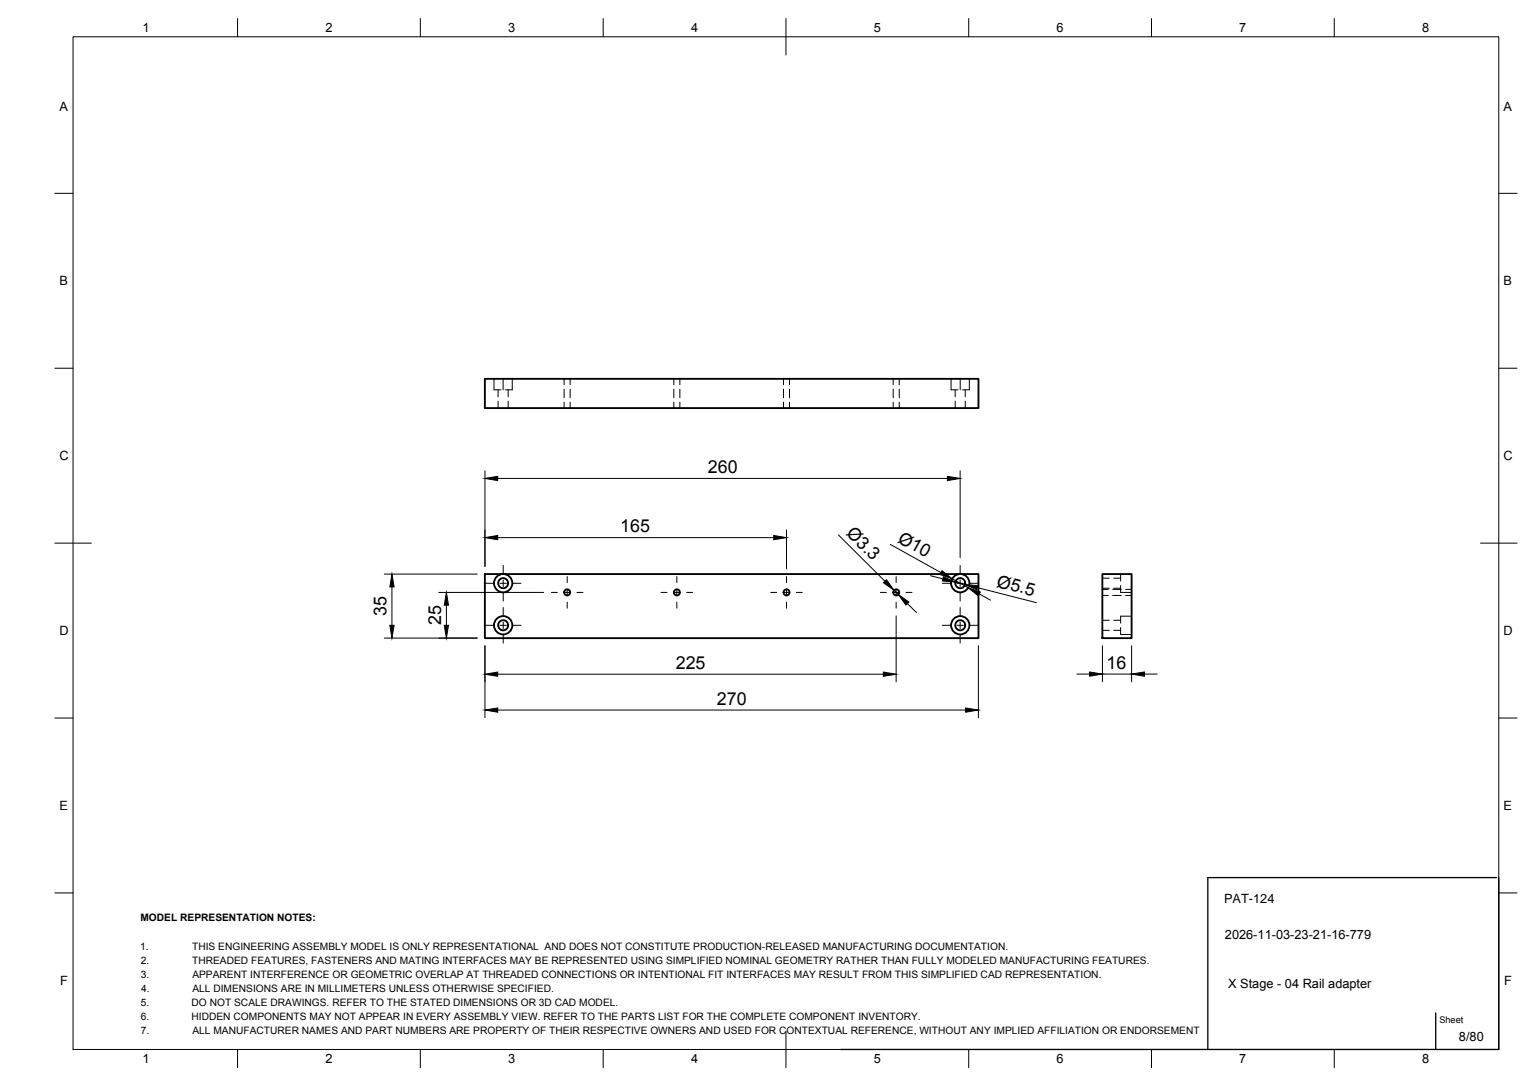
ISO-10303-21;
HEADER;
/* Generated by software containing ST-Developer
 * from STEP Tools, Inc. (www.steptools.com) 
 */

FILE_DESCRIPTION(
/* description */ ('XY cross-slide table'),
/* implementation_level */ '2;1');

FILE_NAME(
/* name */ 'X Stage - 04 Rail adapter.step',
/* time_stamp */ '2026-10-28T03:22:46-07:00',
/* author */ (''),
/* organization */ (''),
/* preprocessor_version */ 'ST-DEVELOPER v20.2',
/* originating_system */ 'Autodesk Translation Framework v15.17.0.0',
/* authorisation */ '');

FILE_SCHEMA (('AUTOMOTIVE_DESIGN { 1 0 10303 214 3 1 1 }'));
ENDSEC;

DATA;
#10=MECHANICAL_DESIGN_GEOMETRIC_PRESENTATION_REPRESENTATION('',(#1673),#62984);
#1507=SHAPE_REPRESENTATION_RELATIONSHIP('SRR','None',#63355,#1590);
#1590=ADVANCED_BREP_SHAPE_REPRESENTATION('',(#1786),#62892);
#1673=STYLED_ITEM('',(#63898),#1786);
#1786=MANIFOLD_SOLID_BREP('Body1',#22967);
#1907=FACE_BOUND('',#4239,.T.);
#1908=FACE_BOUND('',#4242,.T.);
#1909=FACE_BOUND('',#4245,.T.);
#1910=FACE_BOUND('',#4248,.T.);
#1911=FACE_BOUND('',#4250,.T.);
#1912=FACE_BOUND('',#4251,.T.);
#1913=FACE_BOUND('',#4252,.T.);
#1914=FACE_BOUND('',#4253,.T.);
#1915=FACE_BOUND('',#4254,.T.);
#1916=FACE_BOUND('',#4255,.T.);
#1917=FACE_BOUND('',#4265,.T.);
#1918=FACE_BOUND('',#4266,.T.);
#1919=FACE_BOUND('',#4267,.T.);
#1920=FACE_BOUND('',#4268,.T.);
#1921=FACE_BOUND('',#4269,.T.);
#1922=FACE_BOUND('',#4270,.T.);
#1923=FACE_BOUND('',#4271,.T.);
#1924=FACE_BOUND('',#4272,.T.);
#2314=PLANE('',#24076);
#2315=PLANE('',#24081);
#2316=PLANE('',#24086);
#2317=PLANE('',#24091);
#2318=PLANE('',#24093);
#2319=PLANE('',#24102);
#2320=PLANE('',#24103);
#2321=PLANE('',#24104);
#2322=PLANE('',#24105);
#2323=PLANE('',#24106);
#2897=FACE_OUTER_BOUND('',#4231,.T.);
#2898=FACE_OUTER_BOUND('',#4232,.T.);
#2899=FACE_OUTER_BOUND('',#4233,.T.);
#2900=FACE_OUTER_BOUND('',#4234,.T.);
#2901=FACE_OUTER_BOUND('',#4235,.T.);
#2902=FACE_OUTER_BOUND('',#4236,.T.);
#2903=FACE_OUTER_BOUND('',#4237,.T.);
#2904=FACE_OUTER_BOUND('',#4238,.T.);
#2905=FACE_OUTER_BOUND('',#4240,.T.);
#2906=FACE_OUTER_BOUND('',#4241,.T.);
#2907=FACE_OUTER_BOUND('',#4243,.T.);
#2908=FACE_OUTER_BOUND('',#4244,.T.);
#2909=FACE_OUTER_BOUND('',#4246,.T.);
#2910=FACE_OUTER_BOUND('',#4247,.T.);
#2911=FACE_OUTER_BOUND('',#4249,.T.);
#2912=FACE_OUTER_BOUND('',#4256,.T.);
#2913=FACE_OUTER_BOUND('',#4257,.T.);
#2914=FACE_OUTER_BOUND('',#4258,.T.);
#2915=FACE_OUTER_BOUND('',#4259,.T.);
#2916=FACE_OUTER_BOUND('',#4260,.T.);
#2917=FACE_OUTER_BOUND('',#4261,.T.);
#2918=FACE_OUTER_BOUND('',#4262,.T.);
#2919=FACE_OUTER_BOUND('',#4263,.T.);
#2920=FACE_OUTER_BOUND('',#4264,.T.);
#4231=EDGE_LOOP('',(#15036,#15037,#15038,#15039));
#4232=EDGE_LOOP('',(#15040,#15041,#15042,#15043));
#4233=EDGE_LOOP('',(#15044,#15045,#15046,#15047));
#4234=EDGE_LOOP('',(#15048,#15049,#15050,#15051));
#4235=EDGE_LOOP('',(#15052,#15053,#15054,#15055));
#4236=EDGE_LOOP('',(#15056,#15057,#15058,#15059));
#4237=EDGE_LOOP('',(#15060,#15061,#15062,#15063));
#4238=EDGE_LOOP('',(#15064));
#4239=EDGE_LOOP('',(#15065));
#4240=EDGE_LOOP('',(#15066,#15067,#15068,#15069));
#4241=EDGE_LOOP('',(#15070,#15071));
#4242=EDGE_LOOP('',(#15072));
#4243=EDGE_LOOP('',(#15073,#15074,#15075,#15076));
#4244=EDGE_LOOP('',(#15077));
#4245=EDGE_LOOP('',(#15078));
#4246=EDGE_LOOP('',(#15079,#15080,#15081,#15082));
#4247=EDGE_LOOP('',(#15083,#15084));
#4248=EDGE_LOOP('',(#15085));
#4249=EDGE_LOOP('',(#15086,#15087,#15088,#15089,#15090,#15091,#15092,#15093,
#15094,#15095));
#4250=EDGE_LOOP('',(#15096));
#4251=EDGE_LOOP('',(#15097));
#4252=EDGE_LOOP('',(#15098));
#4253=EDGE_LOOP('',(#15099));
#4254=EDGE_LOOP('',(#15100));
#4255=EDGE_LOOP('',(#15101));
#4256=EDGE_LOOP('',(#15102,#15103,#15104,#15105));
#4257=EDGE_LOOP('',(#15106,#15107,#15108,#15109));
#4258=EDGE_LOOP('',(#15110,#15111,#15112,#15113));
#4259=EDGE_LOOP('',(#15114,#15115,#15116,#15117));
#4260=EDGE_LOOP('',(#15118,#15119,#15120,#15121,#15122,#15123,#15124,#15125,
#15126,#15127));
#4261=EDGE_LOOP('',(#15128,#15129,#15130,#15131));
#4262=EDGE_LOOP('',(#15132,#15133,#15134,#15135));
#4263=EDGE_LOOP('',(#15136,#15137,#15138,#15139));
#4264=EDGE_LOOP('',(#15140,#15141,#15142,#15143));
#4265=EDGE_LOOP('',(#15144));
#4266=EDGE_LOOP('',(#15145));
#4267=EDGE_LOOP('',(#15146));
#4268=EDGE_LOOP('',(#15147));
#4269=EDGE_LOOP('',(#15148));
#4270=EDGE_LOOP('',(#15149));
#4271=EDGE_LOOP('',(#15150));
#4272=EDGE_LOOP('',(#15151));
#5952=LINE('',#33018,#7439);
#5953=LINE('',#33022,#7440);
#5954=LINE('',#33027,#7441);
#5955=LINE('',#33031,#7442);
#5956=LINE('',#33037,#7443);
#5957=LINE('',#33043,#7444);
#5958=LINE('',#33049,#7445);
#5959=LINE('',#33055,#7446);
#5960=LINE('',#33061,#7447);
#5961=LINE('',#33068,#7448);
#5962=LINE('',#33077,#7449);
#5963=LINE('',#33084,#7450);
#5964=LINE('',#33092,#7451);
#5965=LINE('',#33094,#7452);
#5966=LINE('',#33096,#7453);
#5967=LINE('',#33097,#7454);
#5968=LINE('',#33098,#7455);
#5969=LINE('',#33099,#7456);
#5970=LINE('',#33103,#7457);
#5971=LINE('',#33107,#7458);
#5972=LINE('',#33111,#7459);
#5973=LINE('',#33115,#7460);
#5974=LINE('',#33119,#7461);
#5975=LINE('',#33120,#7462);
#5976=LINE('',#33121,#7463);
#5977=LINE('',#33124,#7464);
#5978=LINE('',#33125,#7465);
#5979=LINE('',#33128,#7466);
#5980=LINE('',#33129,#7467);
#5981=LINE('',#33131,#7468);
#7439=VECTOR('',#26619,0.5);
#7440=VECTOR('',#26622,1.);
#7441=VECTOR('',#26627,0.5);
#7442=VECTOR('',#26630,1.);
#7443=VECTOR('',#26637,0.164999999999999);
#7444=VECTOR('',#26644,0.164999999999999);
#7445=VECTOR('',#26651,0.165);
#7446=VECTOR('',#26658,0.164999999999999);
#7447=VECTOR('',#26665,0.5);
#7448=VECTOR('',#26676,1.);
#7449=VECTOR('',#26687,0.5);
#7450=VECTOR('',#26698,1.);
#7451=VECTOR('',#26707,1.);
#7452=VECTOR('',#26708,1.);
#7453=VECTOR('',#26709,1.);
#7454=VECTOR('',#26710,1.);
#7455=VECTOR('',#26711,1.);
#7456=VECTOR('',#26712,1.);
#7457=VECTOR('',#26717,0.274999999999999);
#7458=VECTOR('',#26722,0.275);
#7459=VECTOR('',#26727,0.275);
#7460=VECTOR('',#26732,0.274999999999999);
#7461=VECTOR('',#26735,1.);
#7462=VECTOR('',#26736,1.);
#7463=VECTOR('',#26737,1.);
#7464=VECTOR('',#26740,1.);
#7465=VECTOR('',#26741,1.);
#7466=VECTOR('',#26744,1.);
#7467=VECTOR('',#26745,1.);
#7468=VECTOR('',#26748,1.);
#8900=CIRCLE('',#24056,0.5);
#8901=CIRCLE('',#24057,0.5);
#8902=CIRCLE('',#24059,0.5);
#8903=CIRCLE('',#24060,0.5);
#8904=CIRCLE('',#24062,0.164999999999999);
#8905=CIRCLE('',#24063,0.164999999999999);
#8906=CIRCLE('',#24065,0.164999999999999);
#8907=CIRCLE('',#24066,0.164999999999999);
#8908=CIRCLE('',#24068,0.165);
#8909=CIRCLE('',#24069,0.165);
#8910=CIRCLE('',#24071,0.164999999999999);
#8911=CIRCLE('',#24072,0.164999999999999);
#8912=CIRCLE('',#24074,0.5);
#8913=CIRCLE('',#24075,0.5);
#8914=CIRCLE('',#24077,0.274999999999999);
#8915=CIRCLE('',#24079,0.5);
#8916=CIRCLE('',#24080,0.5);
#8917=CIRCLE('',#24082,0.275);
#8918=CIRCLE('',#24084,0.5);
#8919=CIRCLE('',#24085,0.5);
#8920=CIRCLE('',#24087,0.275);
#8921=CIRCLE('',#24089,0.5);
#8922=CIRCLE('',#24090,0.5);
#8923=CIRCLE('',#24092,0.274999999999999);
#8924=CIRCLE('',#24095,0.274999999999999);
#8925=CIRCLE('',#24097,0.275);
#8926=CIRCLE('',#24099,0.275);
#8927=CIRCLE('',#24101,0.274999999999999);
#9817=VERTEX_POINT('',#33016);
#9818=VERTEX_POINT('',#33017);
#9819=VERTEX_POINT('',#33019);
#9820=VERTEX_POINT('',#33021);
#9821=VERTEX_POINT('',#33025);
#9822=VERTEX_POINT('',#33026);
#9823=VERTEX_POINT('',#33028);
#9824=VERTEX_POINT('',#33030);
#9825=VERTEX_POINT('',#33034);
#9826=VERTEX_POINT('',#33036);
#9827=VERTEX_POINT('',#33040);
#9828=VERTEX_POINT('',#33042);
#9829=VERTEX_POINT('',#33046);
#9830=VERTEX_POINT('',#33048);
#9831=VERTEX_POINT('',#33052);
#9832=VERTEX_POINT('',#33054);
#9833=VERTEX_POINT('',#33058);
#9834=VERTEX_POINT('',#33060);
#9835=VERTEX_POINT('',#33064);
#9836=VERTEX_POINT('',#33071);
#9837=VERTEX_POINT('',#33074);
#9838=VERTEX_POINT('',#33076);
#9839=VERTEX_POINT('',#33080);
#9840=VERTEX_POINT('',#33087);
#9841=VERTEX_POINT('',#33090);
#9842=VERTEX_POINT('',#33091);
#9843=VERTEX_POINT('',#33093);
#9844=VERTEX_POINT('',#33095);
#9845=VERTEX_POINT('',#33101);
#9846=VERTEX_POINT('',#33105);
#9847=VERTEX_POINT('',#33109);
#9848=VERTEX_POINT('',#33113);
#9849=VERTEX_POINT('',#33117);
#9850=VERTEX_POINT('',#33118);
#9851=VERTEX_POINT('',#33123);
#9852=VERTEX_POINT('',#33127);
#11902=EDGE_CURVE('',#9817,#9818,#5952,.T.);
#11903=EDGE_CURVE('',#9819,#9817,#8900,.T.);
#11904=EDGE_CURVE('',#9819,#9820,#5953,.T.);
#11905=EDGE_CURVE('',#9818,#9820,#8901,.T.);
#11906=EDGE_CURVE('',#9821,#9822,#5954,.T.);
#11907=EDGE_CURVE('',#9823,#9821,#8902,.T.);
#11908=EDGE_CURVE('',#9823,#9824,#5955,.T.);
#11909=EDGE_CURVE('',#9822,#9824,#8903,.T.);
#11910=EDGE_CURVE('',#9825,#9825,#8904,.T.);
#11911=EDGE_CURVE('',#9825,#9826,#5956,.T.);
#11912=EDGE_CURVE('',#9826,#9826,#8905,.T.);
#11913=EDGE_CURVE('',#9827,#9827,#8906,.T.);
#11914=EDGE_CURVE('',#9827,#9828,#5957,.T.);
#11915=EDGE_CURVE('',#9828,#9828,#8907,.T.);
#11916=EDGE_CURVE('',#9829,#9829,#8908,.T.);
#11917=EDGE_CURVE('',#9829,#9830,#5958,.T.);
#11918=EDGE_CURVE('',#9830,#9830,#8909,.T.);
#11919=EDGE_CURVE('',#9831,#9831,#8910,.T.);
#11920=EDGE_CURVE('',#9831,#9832,#5959,.T.);
#11921=EDGE_CURVE('',#9832,#9832,#8911,.T.);
#11922=EDGE_CURVE('',#9833,#9833,#8912,.T.);
#11923=EDGE_CURVE('',#9833,#9834,#5960,.T.);
#11924=EDGE_CURVE('',#9834,#9834,#8913,.T.);
#11925=EDGE_CURVE('',#9835,#9835,#8914,.T.);
#11926=EDGE_CURVE('',#9824,#9822,#8915,.T.);
#11927=EDGE_CURVE('',#9823,#9824,#5961,.T.);
#11928=EDGE_CURVE('',#9821,#9823,#8916,.T.);
#11929=EDGE_CURVE('',#9836,#9836,#8917,.T.);
#11930=EDGE_CURVE('',#9837,#9837,#8918,.T.);
#11931=EDGE_CURVE('',#9837,#9838,#5962,.T.);
#11932=EDGE_CURVE('',#9838,#9838,#8919,.T.);
#11933=EDGE_CURVE('',#9839,#9839,#8920,.T.);
#11934=EDGE_CURVE('',#9820,#9818,#8921,.T.);
#11935=EDGE_CURVE('',#9819,#9820,#5963,.T.);
#11936=EDGE_CURVE('',#9817,#9819,#8922,.T.);
#11937=EDGE_CURVE('',#9840,#9840,#8923,.T.);
#11938=EDGE_CURVE('',#9841,#9842,#5964,.T.);
#11939=EDGE_CURVE('',#9842,#9843,#5965,.T.);
#11940=EDGE_CURVE('',#9843,#9844,#5966,.T.);
#11941=EDGE_CURVE('',#9844,#9820,#5967,.T.);
#11942=EDGE_CURVE('',#9820,#9824,#5968,.T.);
#11943=EDGE_CURVE('',#9824,#9841,#5969,.T.);
#11944=EDGE_CURVE('',#9845,#9845,#8924,.T.);
#11945=EDGE_CURVE('',#9845,#9835,#5970,.T.);
#11946=EDGE_CURVE('',#9846,#9846,#8925,.T.);
#11947=EDGE_CURVE('',#9846,#9836,#5971,.T.);
#11948=EDGE_CURVE('',#9847,#9847,#8926,.T.);
#11949=EDGE_CURVE('',#9847,#9839,#5972,.T.);
#11950=EDGE_CURVE('',#9848,#9848,#8927,.T.);
#11951=EDGE_CURVE('',#9848,#9840,#5973,.T.);
#11952=EDGE_CURVE('',#9849,#9850,#5974,.T.);
#11953=EDGE_CURVE('',#9850,#9841,#5975,.T.);
#11954=EDGE_CURVE('',#9849,#9844,#5976,.T.);
#11955=EDGE_CURVE('',#9851,#9849,#5977,.T.);
#11956=EDGE_CURVE('',#9851,#9843,#5978,.T.);
#11957=EDGE_CURVE('',#9852,#9851,#5979,.T.);
#11958=EDGE_CURVE('',#9852,#9842,#5980,.T.);
#11959=EDGE_CURVE('',#9850,#9852,#5981,.T.);
#15036=ORIENTED_EDGE('',*,*,#11902,.F.);
#15037=ORIENTED_EDGE('',*,*,#11903,.F.);
#15038=ORIENTED_EDGE('',*,*,#11904,.T.);
#15039=ORIENTED_EDGE('',*,*,#11905,.F.);
#15040=ORIENTED_EDGE('',*,*,#11906,.F.);
#15041=ORIENTED_EDGE('',*,*,#11907,.F.);
#15042=ORIENTED_EDGE('',*,*,#11908,.T.);
#15043=ORIENTED_EDGE('',*,*,#11909,.F.);
#15044=ORIENTED_EDGE('',*,*,#11910,.F.);
#15045=ORIENTED_EDGE('',*,*,#11911,.T.);
#15046=ORIENTED_EDGE('',*,*,#11912,.F.);
#15047=ORIENTED_EDGE('',*,*,#11911,.F.);
#15048=ORIENTED_EDGE('',*,*,#11913,.F.);
#15049=ORIENTED_EDGE('',*,*,#11914,.T.);
#15050=ORIENTED_EDGE('',*,*,#11915,.F.);
#15051=ORIENTED_EDGE('',*,*,#11914,.F.);
#15052=ORIENTED_EDGE('',*,*,#11916,.F.);
#15053=ORIENTED_EDGE('',*,*,#11917,.T.);
#15054=ORIENTED_EDGE('',*,*,#11918,.F.);
#15055=ORIENTED_EDGE('',*,*,#11917,.F.);
#15056=ORIENTED_EDGE('',*,*,#11919,.F.);
#15057=ORIENTED_EDGE('',*,*,#11920,.T.);
#15058=ORIENTED_EDGE('',*,*,#11921,.F.);
#15059=ORIENTED_EDGE('',*,*,#11920,.F.);
#15060=ORIENTED_EDGE('',*,*,#11922,.F.);
#15061=ORIENTED_EDGE('',*,*,#11923,.T.);
#15062=ORIENTED_EDGE('',*,*,#11924,.F.);
#15063=ORIENTED_EDGE('',*,*,#11923,.F.);
#15064=ORIENTED_EDGE('',*,*,#11922,.T.);
#15065=ORIENTED_EDGE('',*,*,#11925,.F.);
#15066=ORIENTED_EDGE('',*,*,#11906,.T.);
#15067=ORIENTED_EDGE('',*,*,#11926,.F.);
#15068=ORIENTED_EDGE('',*,*,#11927,.F.);
#15069=ORIENTED_EDGE('',*,*,#11928,.F.);
#15070=ORIENTED_EDGE('',*,*,#11907,.T.);
#15071=ORIENTED_EDGE('',*,*,#11928,.T.);
#15072=ORIENTED_EDGE('',*,*,#11929,.F.);
#15073=ORIENTED_EDGE('',*,*,#11930,.F.);
#15074=ORIENTED_EDGE('',*,*,#11931,.T.);
#15075=ORIENTED_EDGE('',*,*,#11932,.F.);
#15076=ORIENTED_EDGE('',*,*,#11931,.F.);
#15077=ORIENTED_EDGE('',*,*,#11930,.T.);
#15078=ORIENTED_EDGE('',*,*,#11933,.F.);
#15079=ORIENTED_EDGE('',*,*,#11902,.T.);
#15080=ORIENTED_EDGE('',*,*,#11934,.F.);
#15081=ORIENTED_EDGE('',*,*,#11935,.F.);
#15082=ORIENTED_EDGE('',*,*,#11936,.F.);
#15083=ORIENTED_EDGE('',*,*,#11903,.T.);
#15084=ORIENTED_EDGE('',*,*,#11936,.T.);
#15085=ORIENTED_EDGE('',*,*,#11937,.F.);
#15086=ORIENTED_EDGE('',*,*,#11938,.T.);
#15087=ORIENTED_EDGE('',*,*,#11939,.T.);
#15088=ORIENTED_EDGE('',*,*,#11940,.T.);
#15089=ORIENTED_EDGE('',*,*,#11941,.T.);
#15090=ORIENTED_EDGE('',*,*,#11934,.T.);
#15091=ORIENTED_EDGE('',*,*,#11905,.T.);
#15092=ORIENTED_EDGE('',*,*,#11942,.T.);
#15093=ORIENTED_EDGE('',*,*,#11926,.T.);
#15094=ORIENTED_EDGE('',*,*,#11909,.T.);
#15095=ORIENTED_EDGE('',*,*,#11943,.T.);
#15096=ORIENTED_EDGE('',*,*,#11924,.T.);
#15097=ORIENTED_EDGE('',*,*,#11932,.T.);
#15098=ORIENTED_EDGE('',*,*,#11921,.T.);
#15099=ORIENTED_EDGE('',*,*,#11918,.T.);
#15100=ORIENTED_EDGE('',*,*,#11915,.T.);
#15101=ORIENTED_EDGE('',*,*,#11912,.T.);
#15102=ORIENTED_EDGE('',*,*,#11944,.F.);
#15103=ORIENTED_EDGE('',*,*,#11945,.T.);
#15104=ORIENTED_EDGE('',*,*,#11925,.T.);
#15105=ORIENTED_EDGE('',*,*,#11945,.F.);
#15106=ORIENTED_EDGE('',*,*,#11946,.F.);
#15107=ORIENTED_EDGE('',*,*,#11947,.T.);
#15108=ORIENTED_EDGE('',*,*,#11929,.T.);
#15109=ORIENTED_EDGE('',*,*,#11947,.F.);
#15110=ORIENTED_EDGE('',*,*,#11948,.F.);
#15111=ORIENTED_EDGE('',*,*,#11949,.T.);
#15112=ORIENTED_EDGE('',*,*,#11933,.T.);
#15113=ORIENTED_EDGE('',*,*,#11949,.F.);
#15114=ORIENTED_EDGE('',*,*,#11950,.F.);
#15115=ORIENTED_EDGE('',*,*,#11951,.T.);
#15116=ORIENTED_EDGE('',*,*,#11937,.T.);
#15117=ORIENTED_EDGE('',*,*,#11951,.F.);
#15118=ORIENTED_EDGE('',*,*,#11952,.T.);
#15119=ORIENTED_EDGE('',*,*,#11953,.T.);
#15120=ORIENTED_EDGE('',*,*,#11943,.F.);
#15121=ORIENTED_EDGE('',*,*,#11908,.F.);
#15122=ORIENTED_EDGE('',*,*,#11927,.T.);
#15123=ORIENTED_EDGE('',*,*,#11942,.F.);
#15124=ORIENTED_EDGE('',*,*,#11904,.F.);
#15125=ORIENTED_EDGE('',*,*,#11935,.T.);
#15126=ORIENTED_EDGE('',*,*,#11941,.F.);
#15127=ORIENTED_EDGE('',*,*,#11954,.F.);
#15128=ORIENTED_EDGE('',*,*,#11955,.T.);
#15129=ORIENTED_EDGE('',*,*,#11954,.T.);
#15130=ORIENTED_EDGE('',*,*,#11940,.F.);
#15131=ORIENTED_EDGE('',*,*,#11956,.F.);
#15132=ORIENTED_EDGE('',*,*,#11957,.T.);
#15133=ORIENTED_EDGE('',*,*,#11956,.T.);
#15134=ORIENTED_EDGE('',*,*,#11939,.F.);
#15135=ORIENTED_EDGE('',*,*,#11958,.F.);
#15136=ORIENTED_EDGE('',*,*,#11959,.T.);
#15137=ORIENTED_EDGE('',*,*,#11958,.T.);
#15138=ORIENTED_EDGE('',*,*,#11938,.F.);
#15139=ORIENTED_EDGE('',*,*,#11953,.F.);
#15140=ORIENTED_EDGE('',*,*,#11959,.F.);
#15141=ORIENTED_EDGE('',*,*,#11952,.F.);
#15142=ORIENTED_EDGE('',*,*,#11955,.F.);
#15143=ORIENTED_EDGE('',*,*,#11957,.F.);
#15144=ORIENTED_EDGE('',*,*,#11950,.T.);
#15145=ORIENTED_EDGE('',*,*,#11948,.T.);
#15146=ORIENTED_EDGE('',*,*,#11946,.T.);
#15147=ORIENTED_EDGE('',*,*,#11944,.T.);
#15148=ORIENTED_EDGE('',*,*,#11919,.T.);
#15149=ORIENTED_EDGE('',*,*,#11916,.T.);
#15150=ORIENTED_EDGE('',*,*,#11913,.T.);
#15151=ORIENTED_EDGE('',*,*,#11910,.T.);
#21050=CYLINDRICAL_SURFACE('',#24055,0.5);
#21051=CYLINDRICAL_SURFACE('',#24058,0.5);
#21052=CYLINDRICAL_SURFACE('',#24061,0.164999999999999);
#21053=CYLINDRICAL_SURFACE('',#24064,0.164999999999999);
#21054=CYLINDRICAL_SURFACE('',#24067,0.165);
#21055=CYLINDRICAL_SURFACE('',#24070,0.164999999999999);
#21056=CYLINDRICAL_SURFACE('',#24073,0.5);
#21057=CYLINDRICAL_SURFACE('',#24078,0.5);
#21058=CYLINDRICAL_SURFACE('',#24083,0.5);
#21059=CYLINDRICAL_SURFACE('',#24088,0.5);
#21060=CYLINDRICAL_SURFACE('',#24094,0.274999999999999);
#21061=CYLINDRICAL_SURFACE('',#24096,0.275);
#21062=CYLINDRICAL_SURFACE('',#24098,0.275);
#21063=CYLINDRICAL_SURFACE('',#24100,0.274999999999999);
#21678=ADVANCED_FACE('',(#2897),#21050,.F.);
#21679=ADVANCED_FACE('',(#2898),#21051,.F.);
#21680=ADVANCED_FACE('',(#2899),#21052,.F.);
#21681=ADVANCED_FACE('',(#2900),#21053,.F.);
#21682=ADVANCED_FACE('',(#2901),#21054,.F.);
#21683=ADVANCED_FACE('',(#2902),#21055,.F.);
#21684=ADVANCED_FACE('',(#2903),#21056,.F.);
#21685=ADVANCED_FACE('',(#2904,#1907),#2314,.T.);
#21686=ADVANCED_FACE('',(#2905),#21057,.F.);
#21687=ADVANCED_FACE('',(#2906,#1908),#2315,.T.);
#21688=ADVANCED_FACE('',(#2907),#21058,.F.);
#21689=ADVANCED_FACE('',(#2908,#1909),#2316,.T.);
#21690=ADVANCED_FACE('',(#2909),#21059,.F.);
#21691=ADVANCED_FACE('',(#2910,#1910),#2317,.T.);
#21692=ADVANCED_FACE('',(#2911,#1911,#1912,#1913,#1914,#1915,#1916),#2318,
 .T.);
#21693=ADVANCED_FACE('',(#2912),#21060,.F.);
#21694=ADVANCED_FACE('',(#2913),#21061,.F.);
#21695=ADVANCED_FACE('',(#2914),#21062,.F.);
#21696=ADVANCED_FACE('',(#2915),#21063,.F.);
#21697=ADVANCED_FACE('',(#2916),#2319,.T.);
#21698=ADVANCED_FACE('',(#2917),#2320,.T.);
#21699=ADVANCED_FACE('',(#2918),#2321,.T.);
#21700=ADVANCED_FACE('',(#2919),#2322,.T.);
#21701=ADVANCED_FACE('',(#2920,#1917,#1918,#1919,#1920,#1921,#1922,#1923,
#1924),#2323,.F.);
#22967=CLOSED_SHELL('',(#21678,#21679,#21680,#21681,#21682,#21683,#21684,
#21685,#21686,#21687,#21688,#21689,#21690,#21691,#21692,#21693,#21694,#21695,
#21696,#21697,#21698,#21699,#21700,#21701));
#24054=AXIS2_PLACEMENT_3D('',#33014,#26615,#26616);
#24055=AXIS2_PLACEMENT_3D('',#33015,#26617,#26618);
#24056=AXIS2_PLACEMENT_3D('',#33020,#26620,#26621);
#24057=AXIS2_PLACEMENT_3D('',#33023,#26623,#26624);
#24058=AXIS2_PLACEMENT_3D('',#33024,#26625,#26626);
#24059=AXIS2_PLACEMENT_3D('',#33029,#26628,#26629);
#24060=AXIS2_PLACEMENT_3D('',#33032,#26631,#26632);
#24061=AXIS2_PLACEMENT_3D('',#33033,#26633,#26634);
#24062=AXIS2_PLACEMENT_3D('',#33035,#26635,#26636);
#24063=AXIS2_PLACEMENT_3D('',#33038,#26638,#26639);
#24064=AXIS2_PLACEMENT_3D('',#33039,#26640,#26641);
#24065=AXIS2_PLACEMENT_3D('',#33041,#26642,#26643);
#24066=AXIS2_PLACEMENT_3D('',#33044,#26645,#26646);
#24067=AXIS2_PLACEMENT_3D('',#33045,#26647,#26648);
#24068=AXIS2_PLACEMENT_3D('',#33047,#26649,#26650);
#24069=AXIS2_PLACEMENT_3D('',#33050,#26652,#26653);
#24070=AXIS2_PLACEMENT_3D('',#33051,#26654,#26655);
#24071=AXIS2_PLACEMENT_3D('',#33053,#26656,#26657);
#24072=AXIS2_PLACEMENT_3D('',#33056,#26659,#26660);
#24073=AXIS2_PLACEMENT_3D('',#33057,#26661,#26662);
#24074=AXIS2_PLACEMENT_3D('',#33059,#26663,#26664);
#24075=AXIS2_PLACEMENT_3D('',#33062,#26666,#26667);
#24076=AXIS2_PLACEMENT_3D('',#33063,#26668,#26669);
#24077=AXIS2_PLACEMENT_3D('',#33065,#26670,#26671);
#24078=AXIS2_PLACEMENT_3D('',#33066,#26672,#26673);
#24079=AXIS2_PLACEMENT_3D('',#33067,#26674,#26675);
#24080=AXIS2_PLACEMENT_3D('',#33069,#26677,#26678);
#24081=AXIS2_PLACEMENT_3D('',#33070,#26679,#26680);
#24082=AXIS2_PLACEMENT_3D('',#33072,#26681,#26682);
#24083=AXIS2_PLACEMENT_3D('',#33073,#26683,#26684);
#24084=AXIS2_PLACEMENT_3D('',#33075,#26685,#26686);
#24085=AXIS2_PLACEMENT_3D('',#33078,#26688,#26689);
#24086=AXIS2_PLACEMENT_3D('',#33079,#26690,#26691);
#24087=AXIS2_PLACEMENT_3D('',#33081,#26692,#26693);
#24088=AXIS2_PLACEMENT_3D('',#33082,#26694,#26695);
#24089=AXIS2_PLACEMENT_3D('',#33083,#26696,#26697);
#24090=AXIS2_PLACEMENT_3D('',#33085,#26699,#26700);
#24091=AXIS2_PLACEMENT_3D('',#33086,#26701,#26702);
#24092=AXIS2_PLACEMENT_3D('',#33088,#26703,#26704);
#24093=AXIS2_PLACEMENT_3D('',#33089,#26705,#26706);
#24094=AXIS2_PLACEMENT_3D('',#33100,#26713,#26714);
#24095=AXIS2_PLACEMENT_3D('',#33102,#26715,#26716);
#24096=AXIS2_PLACEMENT_3D('',#33104,#26718,#26719);
#24097=AXIS2_PLACEMENT_3D('',#33106,#26720,#26721);
#24098=AXIS2_PLACEMENT_3D('',#33108,#26723,#26724);
#24099=AXIS2_PLACEMENT_3D('',#33110,#26725,#26726);
#24100=AXIS2_PLACEMENT_3D('',#33112,#26728,#26729);
#24101=AXIS2_PLACEMENT_3D('',#33114,#26730,#26731);
#24102=AXIS2_PLACEMENT_3D('',#33116,#26733,#26734);
#24103=AXIS2_PLACEMENT_3D('',#33122,#26738,#26739);
#24104=AXIS2_PLACEMENT_3D('',#33126,#26742,#26743);
#24105=AXIS2_PLACEMENT_3D('',#33130,#26746,#26747);
#24106=AXIS2_PLACEMENT_3D('',#33132,#26749,#26750);
#26615=DIRECTION('axis',(0.,0.,1.));
#26616=DIRECTION('refdir',(1.,0.,0.));
#26617=DIRECTION('center_axis',(0.,0.,1.));
#26618=DIRECTION('ref_axis',(1.,0.,0.));
#26619=DIRECTION('',(0.,0.,1.));
#26620=DIRECTION('center_axis',(0.,0.,1.));
#26621=DIRECTION('ref_axis',(1.,0.,0.));
#26622=DIRECTION('',(0.,0.,1.));
#26623=DIRECTION('center_axis',(0.,0.,-1.));
#26624=DIRECTION('ref_axis',(1.,0.,0.));
#26625=DIRECTION('center_axis',(0.,0.,1.));
#26626=DIRECTION('ref_axis',(1.,0.,0.));
#26627=DIRECTION('',(0.,0.,1.));
#26628=DIRECTION('center_axis',(0.,0.,1.));
#26629=DIRECTION('ref_axis',(1.,0.,0.));
#26630=DIRECTION('',(0.,0.,1.));
#26631=DIRECTION('center_axis',(0.,0.,-1.));
#26632=DIRECTION('ref_axis',(1.,0.,0.));
#26633=DIRECTION('center_axis',(0.,0.,1.));
#26634=DIRECTION('ref_axis',(1.,0.,0.));
#26635=DIRECTION('center_axis',(0.,0.,1.));
#26636=DIRECTION('ref_axis',(1.,0.,0.));
#26637=DIRECTION('',(0.,0.,1.));
#26638=DIRECTION('center_axis',(0.,0.,-1.));
#26639=DIRECTION('ref_axis',(1.,0.,0.));
#26640=DIRECTION('center_axis',(0.,0.,1.));
#26641=DIRECTION('ref_axis',(1.,0.,0.));
#26642=DIRECTION('center_axis',(0.,0.,1.));
#26643=DIRECTION('ref_axis',(1.,0.,0.));
#26644=DIRECTION('',(0.,0.,1.));
#26645=DIRECTION('center_axis',(0.,0.,-1.));
#26646=DIRECTION('ref_axis',(1.,0.,0.));
#26647=DIRECTION('center_axis',(0.,0.,1.));
#26648=DIRECTION('ref_axis',(1.,0.,0.));
#26649=DIRECTION('center_axis',(0.,0.,1.));
#26650=DIRECTION('ref_axis',(1.,0.,0.));
#26651=DIRECTION('',(0.,0.,1.));
#26652=DIRECTION('center_axis',(0.,0.,-1.));
#26653=DIRECTION('ref_axis',(1.,0.,0.));
#26654=DIRECTION('center_axis',(0.,0.,1.));
#26655=DIRECTION('ref_axis',(1.,0.,0.));
#26656=DIRECTION('center_axis',(0.,0.,1.));
#26657=DIRECTION('ref_axis',(1.,0.,0.));
#26658=DIRECTION('',(0.,0.,1.));
#26659=DIRECTION('center_axis',(0.,0.,-1.));
#26660=DIRECTION('ref_axis',(1.,0.,0.));
#26661=DIRECTION('center_axis',(0.,0.,1.));
#26662=DIRECTION('ref_axis',(1.,0.,0.));
#26663=DIRECTION('center_axis',(0.,0.,1.));
#26664=DIRECTION('ref_axis',(1.,0.,0.));
#26665=DIRECTION('',(0.,0.,1.));
#26666=DIRECTION('center_axis',(0.,0.,-1.));
#26667=DIRECTION('ref_axis',(1.,0.,0.));
#26668=DIRECTION('center_axis',(0.,0.,1.));
#26669=DIRECTION('ref_axis',(1.,0.,0.));
#26670=DIRECTION('center_axis',(0.,0.,1.));
#26671=DIRECTION('ref_axis',(1.,0.,0.));
#26672=DIRECTION('center_axis',(0.,0.,1.));
#26673=DIRECTION('ref_axis',(1.,0.,0.));
#26674=DIRECTION('center_axis',(0.,0.,-1.));
#26675=DIRECTION('ref_axis',(1.,0.,0.));
#26676=DIRECTION('',(0.,0.,1.));
#26677=DIRECTION('center_axis',(0.,0.,1.));
#26678=DIRECTION('ref_axis',(1.,0.,0.));
#26679=DIRECTION('center_axis',(0.,0.,1.));
#26680=DIRECTION('ref_axis',(1.,0.,0.));
#26681=DIRECTION('center_axis',(0.,0.,1.));
#26682=DIRECTION('ref_axis',(1.,0.,0.));
#26683=DIRECTION('center_axis',(0.,0.,1.));
#26684=DIRECTION('ref_axis',(1.,0.,0.));
#26685=DIRECTION('center_axis',(0.,0.,1.));
#26686=DIRECTION('ref_axis',(1.,0.,0.));
#26687=DIRECTION('',(0.,0.,1.));
#26688=DIRECTION('center_axis',(0.,0.,-1.));
#26689=DIRECTION('ref_axis',(1.,0.,0.));
#26690=DIRECTION('center_axis',(0.,0.,1.));
#26691=DIRECTION('ref_axis',(1.,0.,0.));
#26692=DIRECTION('center_axis',(0.,0.,1.));
#26693=DIRECTION('ref_axis',(1.,0.,0.));
#26694=DIRECTION('center_axis',(0.,0.,1.));
#26695=DIRECTION('ref_axis',(1.,0.,0.));
#26696=DIRECTION('center_axis',(0.,0.,-1.));
#26697=DIRECTION('ref_axis',(1.,0.,0.));
#26698=DIRECTION('',(0.,0.,1.));
#26699=DIRECTION('center_axis',(0.,0.,1.));
#26700=DIRECTION('ref_axis',(1.,0.,0.));
#26701=DIRECTION('center_axis',(0.,0.,1.));
#26702=DIRECTION('ref_axis',(1.,0.,0.));
#26703=DIRECTION('center_axis',(0.,0.,1.));
#26704=DIRECTION('ref_axis',(1.,0.,0.));
#26705=DIRECTION('center_axis',(0.,0.,1.));
#26706=DIRECTION('ref_axis',(1.,0.,0.));
#26707=DIRECTION('',(0.,-1.,0.));
#26708=DIRECTION('',(1.,0.,0.));
#26709=DIRECTION('',(0.,1.,0.));
#26710=DIRECTION('',(-1.,0.,0.));
#26711=DIRECTION('',(-1.,0.,0.));
#26712=DIRECTION('',(-1.,0.,0.));
#26713=DIRECTION('center_axis',(0.,0.,1.));
#26714=DIRECTION('ref_axis',(1.,0.,0.));
#26715=DIRECTION('center_axis',(0.,0.,1.));
#26716=DIRECTION('ref_axis',(1.,0.,0.));
#26717=DIRECTION('',(0.,0.,1.));
#26718=DIRECTION('center_axis',(0.,0.,1.));
#26719=DIRECTION('ref_axis',(1.,0.,0.));
#26720=DIRECTION('center_axis',(0.,0.,1.));
#26721=DIRECTION('ref_axis',(1.,0.,0.));
#26722=DIRECTION('',(0.,0.,1.));
#26723=DIRECTION('center_axis',(0.,0.,1.));
#26724=DIRECTION('ref_axis',(1.,0.,0.));
#26725=DIRECTION('center_axis',(0.,0.,1.));
#26726=DIRECTION('ref_axis',(1.,0.,0.));
#26727=DIRECTION('',(0.,0.,1.));
#26728=DIRECTION('center_axis',(0.,0.,1.));
#26729=DIRECTION('ref_axis',(1.,0.,0.));
#26730=DIRECTION('center_axis',(0.,0.,1.));
#26731=DIRECTION('ref_axis',(1.,0.,0.));
#26732=DIRECTION('',(0.,0.,1.));
#26733=DIRECTION('center_axis',(0.,1.,0.));
#26734=DIRECTION('ref_axis',(-1.,0.,0.));
#26735=DIRECTION('',(-1.,0.,0.));
#26736=DIRECTION('',(0.,0.,1.));
#26737=DIRECTION('',(0.,0.,1.));
#26738=DIRECTION('center_axis',(1.,0.,0.));
#26739=DIRECTION('ref_axis',(0.,1.,0.));
#26740=DIRECTION('',(0.,1.,0.));
#26741=DIRECTION('',(0.,0.,1.));
#26742=DIRECTION('center_axis',(0.,-1.,0.));
#26743=DIRECTION('ref_axis',(1.,0.,0.));
#26744=DIRECTION('',(1.,0.,0.));
#26745=DIRECTION('',(0.,0.,1.));
#26746=DIRECTION('center_axis',(-1.,0.,0.));
#26747=DIRECTION('ref_axis',(0.,-1.,0.));
#26748=DIRECTION('',(0.,-1.,0.));
#26749=DIRECTION('center_axis',(0.,0.,1.));
#26750=DIRECTION('ref_axis',(1.,0.,0.));
#33014=CARTESIAN_POINT('',(0.,0.,0.));
#33015=CARTESIAN_POINT('Origin',(26.,-5.5,2.2));
#33016=CARTESIAN_POINT('',(25.5,-5.5,2.2));
#33017=CARTESIAN_POINT('',(25.5,-5.5,2.8));
#33018=CARTESIAN_POINT('',(25.5,-5.5,2.2));
#33019=CARTESIAN_POINT('',(26.,-5.,2.2));
#33020=CARTESIAN_POINT('Origin',(26.,-5.5,2.2));
#33021=CARTESIAN_POINT('',(26.,-5.,2.8));
#33022=CARTESIAN_POINT('',(26.,-5.,2.2));
#33023=CARTESIAN_POINT('Origin',(26.,-5.5,2.8));
#33024=CARTESIAN_POINT('Origin',(1.,-5.5,2.2));
#33025=CARTESIAN_POINT('',(0.5,-5.5,2.2));
#33026=CARTESIAN_POINT('',(0.5,-5.5,2.8));
#33027=CARTESIAN_POINT('',(0.5,-5.5,2.2));
#33028=CARTESIAN_POINT('',(1.,-5.,2.2));
#33029=CARTESIAN_POINT('Origin',(1.,-5.5,2.2));
#33030=CARTESIAN_POINT('',(1.,-5.,2.8));
#33031=CARTESIAN_POINT('',(1.,-5.,2.2));
#33032=CARTESIAN_POINT('Origin',(1.,-5.5,2.8));
#33033=CARTESIAN_POINT('Origin',(16.5,-6.,1.1));
#33034=CARTESIAN_POINT('',(16.335,-6.,1.2));
#33035=CARTESIAN_POINT('Origin',(16.5,-6.,1.2));
#33036=CARTESIAN_POINT('',(16.335,-6.,2.8));
#33037=CARTESIAN_POINT('',(16.335,-6.,1.1));
#33038=CARTESIAN_POINT('Origin',(16.5,-6.,2.8));
#33039=CARTESIAN_POINT('Origin',(10.5,-6.,1.1));
#33040=CARTESIAN_POINT('',(10.335,-6.,1.2));
#33041=CARTESIAN_POINT('Origin',(10.5,-6.,1.2));
#33042=CARTESIAN_POINT('',(10.335,-6.,2.8));
#33043=CARTESIAN_POINT('',(10.335,-6.,1.1));
#33044=CARTESIAN_POINT('Origin',(10.5,-6.,2.8));
#33045=CARTESIAN_POINT('Origin',(4.5,-6.,1.1));
#33046=CARTESIAN_POINT('',(4.335,-6.,1.2));
#33047=CARTESIAN_POINT('Origin',(4.5,-6.,1.2));
#33048=CARTESIAN_POINT('',(4.335,-6.,2.8));
#33049=CARTESIAN_POINT('',(4.335,-6.,1.1));
#33050=CARTESIAN_POINT('Origin',(4.5,-6.,2.8));
#33051=CARTESIAN_POINT('Origin',(22.5,-6.,1.1));
#33052=CARTESIAN_POINT('',(22.335,-6.,1.2));
#33053=CARTESIAN_POINT('Origin',(22.5,-6.,1.2));
#33054=CARTESIAN_POINT('',(22.335,-6.,2.8));
#33055=CARTESIAN_POINT('',(22.335,-6.,1.1));
#33056=CARTESIAN_POINT('Origin',(22.5,-6.,2.8));
#33057=CARTESIAN_POINT('Origin',(26.,-7.8,2.2));
#33058=CARTESIAN_POINT('',(25.5,-7.8,2.2));
#33059=CARTESIAN_POINT('Origin',(26.,-7.8,2.2));
#33060=CARTESIAN_POINT('',(25.5,-7.8,2.8));
#33061=CARTESIAN_POINT('',(25.5,-7.8,2.2));
#33062=CARTESIAN_POINT('Origin',(26.,-7.8,2.8));
#33063=CARTESIAN_POINT('Origin',(26.,-7.8,2.2));
#33064=CARTESIAN_POINT('',(25.725,-7.8,2.2));
#33065=CARTESIAN_POINT('Origin',(26.,-7.8,2.2));
#33066=CARTESIAN_POINT('Origin',(1.,-5.5,2.2));
#33067=CARTESIAN_POINT('Origin',(1.,-5.5,2.8));
#33068=CARTESIAN_POINT('',(1.,-5.,2.2));
#33069=CARTESIAN_POINT('Origin',(1.,-5.5,2.2));
#33070=CARTESIAN_POINT('Origin',(1.,-5.5,2.2));
#33071=CARTESIAN_POINT('',(0.725,-5.5,2.2));
#33072=CARTESIAN_POINT('Origin',(1.,-5.5,2.2));
#33073=CARTESIAN_POINT('Origin',(1.,-7.8,2.2));
#33074=CARTESIAN_POINT('',(0.5,-7.8,2.2));
#33075=CARTESIAN_POINT('Origin',(1.,-7.8,2.2));
#33076=CARTESIAN_POINT('',(0.5,-7.8,2.8));
#33077=CARTESIAN_POINT('',(0.5,-7.8,2.2));
#33078=CARTESIAN_POINT('Origin',(1.,-7.8,2.8));
#33079=CARTESIAN_POINT('Origin',(1.,-7.8,2.2));
#33080=CARTESIAN_POINT('',(0.725,-7.8,2.2));
#33081=CARTESIAN_POINT('Origin',(1.,-7.8,2.2));
#33082=CARTESIAN_POINT('Origin',(26.,-5.5,2.2));
#33083=CARTESIAN_POINT('Origin',(26.,-5.5,2.8));
#33084=CARTESIAN_POINT('',(26.,-5.,2.2));
#33085=CARTESIAN_POINT('Origin',(26.,-5.5,2.2));
#33086=CARTESIAN_POINT('Origin',(26.,-5.5,2.2));
#33087=CARTESIAN_POINT('',(25.725,-5.5,2.2));
#33088=CARTESIAN_POINT('Origin',(26.,-5.5,2.2));
#33089=CARTESIAN_POINT('Origin',(13.5,-6.75,2.8));
#33090=CARTESIAN_POINT('',(0.,-5.,2.8));
#33091=CARTESIAN_POINT('',(0.,-8.5,2.8));
#33092=CARTESIAN_POINT('',(0.,-5.,2.8));
#33093=CARTESIAN_POINT('',(27.,-8.5,2.8));
#33094=CARTESIAN_POINT('',(0.,-8.5,2.8));
#33095=CARTESIAN_POINT('',(27.,-5.,2.8));
#33096=CARTESIAN_POINT('',(27.,-8.5,2.8));
#33097=CARTESIAN_POINT('',(27.,-5.,2.8));
#33098=CARTESIAN_POINT('',(27.,-5.,2.8));
#33099=CARTESIAN_POINT('',(27.,-5.,2.8));
#33100=CARTESIAN_POINT('Origin',(26.,-7.8,1.1));
#33101=CARTESIAN_POINT('',(25.725,-7.8,1.2));
#33102=CARTESIAN_POINT('Origin',(26.,-7.8,1.2));
#33103=CARTESIAN_POINT('',(25.725,-7.8,1.1));
#33104=CARTESIAN_POINT('Origin',(1.,-5.5,1.1));
#33105=CARTESIAN_POINT('',(0.725,-5.5,1.2));
#33106=CARTESIAN_POINT('Origin',(1.,-5.5,1.2));
#33107=CARTESIAN_POINT('',(0.725,-5.5,1.1));
#33108=CARTESIAN_POINT('Origin',(1.,-7.8,1.1));
#33109=CARTESIAN_POINT('',(0.725,-7.8,1.2));
#33110=CARTESIAN_POINT('Origin',(1.,-7.8,1.2));
#33111=CARTESIAN_POINT('',(0.725,-7.8,1.1));
#33112=CARTESIAN_POINT('Origin',(26.,-5.5,1.1));
#33113=CARTESIAN_POINT('',(25.725,-5.5,1.2));
#33114=CARTESIAN_POINT('Origin',(26.,-5.5,1.2));
#33115=CARTESIAN_POINT('',(25.725,-5.5,1.1));
#33116=CARTESIAN_POINT('Origin',(27.,-5.,1.2));
#33117=CARTESIAN_POINT('',(27.,-5.,1.2));
#33118=CARTESIAN_POINT('',(0.,-5.,1.2));
#33119=CARTESIAN_POINT('',(27.,-5.,1.2));
#33120=CARTESIAN_POINT('',(0.,-5.,1.2));
#33121=CARTESIAN_POINT('',(27.,-5.,1.2));
#33122=CARTESIAN_POINT('Origin',(27.,-8.5,1.2));
#33123=CARTESIAN_POINT('',(27.,-8.5,1.2));
#33124=CARTESIAN_POINT('',(27.,-8.5,1.2));
#33125=CARTESIAN_POINT('',(27.,-8.5,1.2));
#33126=CARTESIAN_POINT('Origin',(0.,-8.5,1.2));
#33127=CARTESIAN_POINT('',(0.,-8.5,1.2));
#33128=CARTESIAN_POINT('',(0.,-8.5,1.2));
#33129=CARTESIAN_POINT('',(0.,-8.5,1.2));
#33130=CARTESIAN_POINT('Origin',(0.,-5.,1.2));
#33131=CARTESIAN_POINT('',(0.,-5.,1.2));
#33132=CARTESIAN_POINT('Origin',(13.5,-6.75,1.2));
#62793=UNCERTAINTY_MEASURE_WITH_UNIT(LENGTH_MEASURE(0.001),#62985,
'DISTANCE_ACCURACY_VALUE',
'Maximum model space distance between geometric entities at asserted c
onnectivities');
#62885=UNCERTAINTY_MEASURE_WITH_UNIT(LENGTH_MEASURE(0.001),#62985,
'DISTANCE_ACCURACY_VALUE',
'Maximum model space distance between geometric entities at asserted c
onnectivities');
#62892=(
GEOMETRIC_REPRESENTATION_CONTEXT(3)
GLOBAL_UNCERTAINTY_ASSIGNED_CONTEXT((#62793))
GLOBAL_UNIT_ASSIGNED_CONTEXT((#62985,#62987,#62988))
REPRESENTATION_CONTEXT('','3D')
);
#62984=(
GEOMETRIC_REPRESENTATION_CONTEXT(3)
GLOBAL_UNCERTAINTY_ASSIGNED_CONTEXT((#62885))
GLOBAL_UNIT_ASSIGNED_CONTEXT((#62985,#62987,#62988))
REPRESENTATION_CONTEXT('','3D')
);
#62985=(
LENGTH_UNIT()
NAMED_UNIT(*)
SI_UNIT(.CENTI.,.METRE.)
);
#62987=(
NAMED_UNIT(*)
PLANE_ANGLE_UNIT()
SI_UNIT($,.RADIAN.)
);
#62988=(
NAMED_UNIT(*)
SI_UNIT($,.STERADIAN.)
SOLID_ANGLE_UNIT()
);
#62995=SHAPE_DEFINITION_REPRESENTATION(#63093,#63355);
#63093=PRODUCT_DEFINITION_SHAPE('',$,#63454);
#63355=SHAPE_REPRESENTATION('',(#24054),#62892);
#63447=PRODUCT_DEFINITION_CONTEXT('part definition',#63743,'design');
#63454=PRODUCT_DEFINITION('X Stage - 04 Rail adapter',
'X Stage - 04 Rail adapter',#63552,#63447);
#63552=PRODUCT_DEFINITION_FORMATION('',$,#63751);
#63743=APPLICATION_CONTEXT(
'Core Data for Automotive Mechanical Design Process');
#63744=PRODUCT_CONTEXT('part definition',#63743,'mechanical');
#63751=PRODUCT('X Stage - 04 Rail adapter','X Stage - 04 Rail adapter',
'X Stage - 04 Rail adapter',(#63744));
#63892=COLOUR_RGB('Light Blue',0.38,0.62,0.78);
#63893=FILL_AREA_STYLE_COLOUR('',#63892);
#63894=FILL_AREA_STYLE('',(#63893));
#63895=SURFACE_STYLE_FILL_AREA(#63894);
#63896=SURFACE_SIDE_STYLE('',(#63895));
#63897=SURFACE_STYLE_USAGE(.BOTH.,#63896);
#63898=PRESENTATION_STYLE_ASSIGNMENT((#63897));
ENDSEC;
END-ISO-10303-21;
